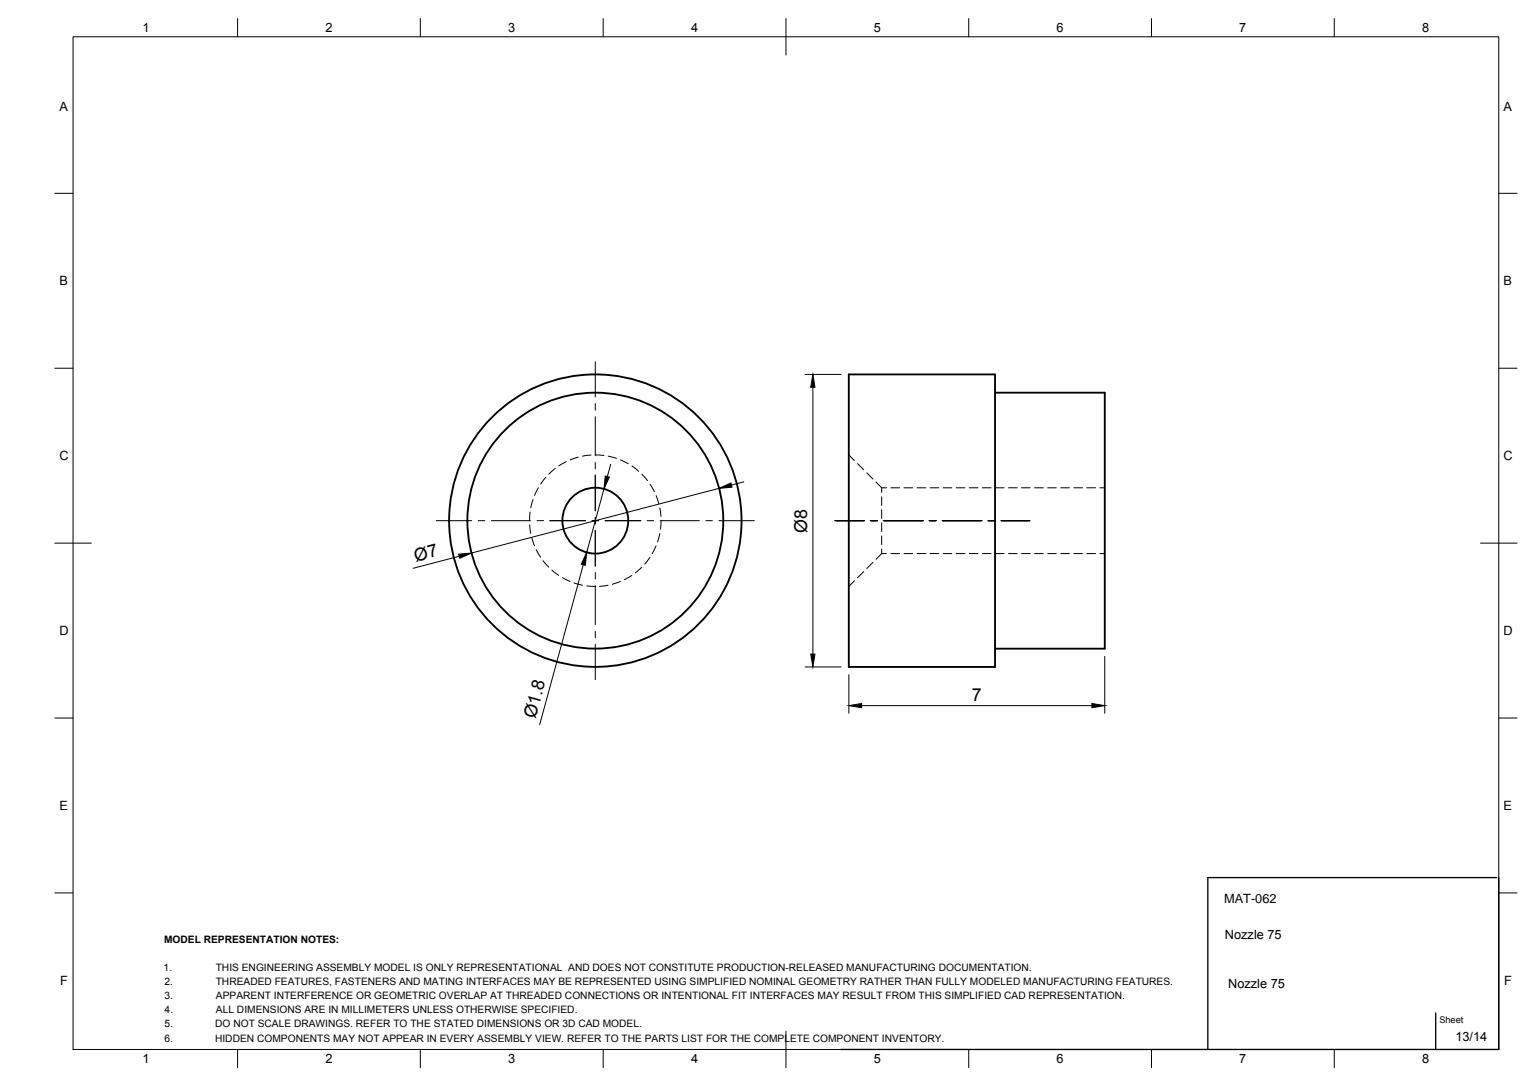
ISO-10303-21;
HEADER;
/* Generated by software containing ST-Developer
 * from STEP Tools, Inc. (www.steptools.com) 
 */

FILE_DESCRIPTION(
/* description */ (''),
/* implementation_level */ '2;1');

FILE_NAME(
/* name */ 'Nozzle 75.step',
/* time_stamp */ '2026-10-24T10:18:25-07:00',
/* author */ (''),
/* organization */ (''),
/* preprocessor_version */ 'ST-DEVELOPER v20.2',
/* originating_system */ 'Autodesk Translation Framework v15.15.0.0',
/* authorisation */ '');

FILE_SCHEMA (('AUTOMOTIVE_DESIGN { 1 0 10303 214 3 1 1 }'));
ENDSEC;

DATA;
#10=MECHANICAL_DESIGN_GEOMETRIC_PRESENTATION_REPRESENTATION('',(#262),#14125);
#196=CONICAL_SURFACE('',#6650,1.80000000000001,0.785398163397454);
#233=SHAPE_REPRESENTATION_RELATIONSHIP('SRR','None',#14207,#243);
#243=ADVANCED_BREP_SHAPE_REPRESENTATION('',(#275),#14121);
#262=STYLED_ITEM('',(#14263),#275);
#275=MANIFOLD_SOLID_BREP('Nozzle 75',#6143);
#560=CYLINDRICAL_SURFACE('',#6640,4.);
#561=CYLINDRICAL_SURFACE('',#6647,0.899999999999989);
#562=CYLINDRICAL_SURFACE('',#6653,3.49999999999993);
#681=FACE_BOUND('',#1362,.T.);
#682=FACE_BOUND('',#1364,.T.);
#683=FACE_BOUND('',#1368,.T.);
#953=FACE_OUTER_BOUND('',#1360,.T.);
#954=FACE_OUTER_BOUND('',#1361,.T.);
#955=FACE_OUTER_BOUND('',#1363,.T.);
#956=FACE_OUTER_BOUND('',#1365,.T.);
#957=FACE_OUTER_BOUND('',#1366,.T.);
#958=FACE_OUTER_BOUND('',#1367,.T.);
#959=FACE_OUTER_BOUND('',#1369,.T.);
#1360=EDGE_LOOP('',(#5025,#5026,#5027,#5028));
#1361=EDGE_LOOP('',(#5029));
#1362=EDGE_LOOP('',(#5030));
#1363=EDGE_LOOP('',(#5031));
#1364=EDGE_LOOP('',(#5032));
#1365=EDGE_LOOP('',(#5033,#5034,#5035,#5036));
#1366=EDGE_LOOP('',(#5037,#5038,#5039,#5040));
#1367=EDGE_LOOP('',(#5041));
#1368=EDGE_LOOP('',(#5042));
#1369=EDGE_LOOP('',(#5043,#5044,#5045,#5046));
#1713=CIRCLE('',#6641,4.);
#1714=CIRCLE('',#6642,4.);
#1715=CIRCLE('',#6644,3.49999999999993);
#1716=CIRCLE('',#6646,1.80000000000001);
#1717=CIRCLE('',#6648,0.900000000000014);
#1718=CIRCLE('',#6649,0.899999999999985);
#1719=CIRCLE('',#6652,3.49999999999993);
#2046=LINE('',#12270,#2434);
#2047=LINE('',#12282,#2435);
#2048=LINE('',#12285,#2436);
#2049=LINE('',#12290,#2437);
#2434=VECTOR('',#7918,4.);
#2435=VECTOR('',#7933,0.899999999999989);
#2436=VECTOR('',#7938,1.80000000000001);
#2437=VECTOR('',#7945,3.49999999999992);
#2930=VERTEX_POINT('',#12267);
#2931=VERTEX_POINT('',#12269);
#2932=VERTEX_POINT('',#12273);
#2933=VERTEX_POINT('',#12276);
#2934=VERTEX_POINT('',#12279);
#2935=VERTEX_POINT('',#12281);
#2936=VERTEX_POINT('',#12287);
#3660=EDGE_CURVE('',#2930,#2930,#1713,.T.);
#3661=EDGE_CURVE('',#2930,#2931,#2046,.T.);
#3662=EDGE_CURVE('',#2931,#2931,#1714,.T.);
#3663=EDGE_CURVE('',#2932,#2932,#1715,.T.);
#3664=EDGE_CURVE('',#2933,#2933,#1716,.T.);
#3665=EDGE_CURVE('',#2934,#2934,#1717,.T.);
#3666=EDGE_CURVE('',#2934,#2935,#2047,.T.);
#3667=EDGE_CURVE('',#2935,#2935,#1718,.T.);
#3668=EDGE_CURVE('',#2935,#2933,#2048,.T.);
#3669=EDGE_CURVE('',#2936,#2936,#1719,.T.);
#3670=EDGE_CURVE('',#2932,#2936,#2049,.T.);
#5025=ORIENTED_EDGE('',*,*,#3660,.T.);
#5026=ORIENTED_EDGE('',*,*,#3661,.T.);
#5027=ORIENTED_EDGE('',*,*,#3662,.F.);
#5028=ORIENTED_EDGE('',*,*,#3661,.F.);
#5029=ORIENTED_EDGE('',*,*,#3662,.T.);
#5030=ORIENTED_EDGE('',*,*,#3663,.F.);
#5031=ORIENTED_EDGE('',*,*,#3660,.F.);
#5032=ORIENTED_EDGE('',*,*,#3664,.F.);
#5033=ORIENTED_EDGE('',*,*,#3665,.T.);
#5034=ORIENTED_EDGE('',*,*,#3666,.T.);
#5035=ORIENTED_EDGE('',*,*,#3667,.T.);
#5036=ORIENTED_EDGE('',*,*,#3666,.F.);
#5037=ORIENTED_EDGE('',*,*,#3667,.F.);
#5038=ORIENTED_EDGE('',*,*,#3668,.T.);
#5039=ORIENTED_EDGE('',*,*,#3664,.T.);
#5040=ORIENTED_EDGE('',*,*,#3668,.F.);
#5041=ORIENTED_EDGE('',*,*,#3669,.T.);
#5042=ORIENTED_EDGE('',*,*,#3665,.F.);
#5043=ORIENTED_EDGE('',*,*,#3663,.T.);
#5044=ORIENTED_EDGE('',*,*,#3670,.T.);
#5045=ORIENTED_EDGE('',*,*,#3669,.F.);
#5046=ORIENTED_EDGE('',*,*,#3670,.F.);
#5722=PLANE('',#6643);
#5723=PLANE('',#6645);
#5724=PLANE('',#6651);
#6002=ADVANCED_FACE('',(#953),#560,.T.);
#6003=ADVANCED_FACE('',(#954,#681),#5722,.T.);
#6004=ADVANCED_FACE('',(#955,#682),#5723,.F.);
#6005=ADVANCED_FACE('',(#956),#561,.F.);
#6006=ADVANCED_FACE('',(#957),#196,.F.);
#6007=ADVANCED_FACE('',(#958,#683),#5724,.T.);
#6008=ADVANCED_FACE('',(#959),#562,.T.);
#6143=CLOSED_SHELL('',(#6002,#6003,#6004,#6005,#6006,#6007,#6008));
#6639=AXIS2_PLACEMENT_3D('',#12265,#7912,#7913);
#6640=AXIS2_PLACEMENT_3D('',#12266,#7914,#7915);
#6641=AXIS2_PLACEMENT_3D('',#12268,#7916,#7917);
#6642=AXIS2_PLACEMENT_3D('',#12271,#7919,#7920);
#6643=AXIS2_PLACEMENT_3D('',#12272,#7921,#7922);
#6644=AXIS2_PLACEMENT_3D('',#12274,#7923,#7924);
#6645=AXIS2_PLACEMENT_3D('',#12275,#7925,#7926);
#6646=AXIS2_PLACEMENT_3D('',#12277,#7927,#7928);
#6647=AXIS2_PLACEMENT_3D('',#12278,#7929,#7930);
#6648=AXIS2_PLACEMENT_3D('',#12280,#7931,#7932);
#6649=AXIS2_PLACEMENT_3D('',#12283,#7934,#7935);
#6650=AXIS2_PLACEMENT_3D('',#12284,#7936,#7937);
#6651=AXIS2_PLACEMENT_3D('',#12286,#7939,#7940);
#6652=AXIS2_PLACEMENT_3D('',#12288,#7941,#7942);
#6653=AXIS2_PLACEMENT_3D('',#12289,#7943,#7944);
#7912=DIRECTION('axis',(0.,0.,1.));
#7913=DIRECTION('refdir',(1.,0.,0.));
#7914=DIRECTION('center_axis',(-0.224143868042018,0.965925826289067,-0.129409522551263));
#7915=DIRECTION('ref_axis',(-0.974116947696296,-0.22604462437946,0.));
#7916=DIRECTION('center_axis',(0.224143868042018,-0.965925826289067,0.129409522551263));
#7917=DIRECTION('ref_axis',(0.974116947696296,0.22604462437946,0.));
#7918=DIRECTION('',(0.224143868042018,-0.965925826289067,0.129409522551263));
#7919=DIRECTION('center_axis',(0.224143868042018,-0.965925826289067,0.129409522551263));
#7920=DIRECTION('ref_axis',(0.974116947696296,0.22604462437946,0.));
#7921=DIRECTION('center_axis',(0.224143868042018,-0.965925826289067,0.129409522551263));
#7922=DIRECTION('ref_axis',(0.,-0.132788176096111,-0.991144439670156));
#7923=DIRECTION('center_axis',(0.224143868042018,-0.965925826289067,0.129409522551263));
#7924=DIRECTION('ref_axis',(0.974116947696296,0.22604462437946,0.));
#7925=DIRECTION('center_axis',(0.224143868042018,-0.965925826289067,0.129409522551263));
#7926=DIRECTION('ref_axis',(0.,-0.132788176096111,-0.991144439670156));
#7927=DIRECTION('center_axis',(-0.224143868042018,0.965925826289067,-0.129409522551263));
#7928=DIRECTION('ref_axis',(-0.974116947696296,-0.22604462437946,0.));
#7929=DIRECTION('center_axis',(-0.224143868042018,0.965925826289067,-0.129409522551263));
#7930=DIRECTION('ref_axis',(-0.974116947696296,-0.22604462437946,0.));
#7931=DIRECTION('center_axis',(0.224143868042018,-0.965925826289067,0.129409522551263));
#7932=DIRECTION('ref_axis',(0.974116947696296,0.22604462437946,0.));
#7933=DIRECTION('',(-0.224143868042018,0.965925826289067,-0.129409522551263));
#7934=DIRECTION('center_axis',(-0.224143868042018,0.965925826289067,-0.129409522551263));
#7935=DIRECTION('ref_axis',(-0.974116947696296,-0.22604462437946,0.));
#7936=DIRECTION('center_axis',(-0.224143868042018,0.965925826289067,-0.129409522551263));
#7937=DIRECTION('ref_axis',(-0.974116947696296,-0.22604462437946,0.));
#7938=DIRECTION('',(0.530311050330904,0.842850388641698,-0.091506350946111));
#7939=DIRECTION('center_axis',(0.224143868042018,-0.965925826289067,0.129409522551263));
#7940=DIRECTION('ref_axis',(0.,-0.132788176096111,-0.991144439670156));
#7941=DIRECTION('center_axis',(0.224143868042018,-0.965925826289067,0.129409522551263));
#7942=DIRECTION('ref_axis',(0.974116947696296,0.22604462437946,0.));
#7943=DIRECTION('center_axis',(-0.224143868042018,0.965925826289067,-0.129409522551263));
#7944=DIRECTION('ref_axis',(-0.974116947696296,-0.22604462437946,0.));
#7945=DIRECTION('',(0.224143868042018,-0.965925826289067,0.129409522551263));
#12265=CARTESIAN_POINT('',(0.,0.,0.));
#12266=CARTESIAN_POINT('Origin',(-88.8998569762207,131.101020514434,-63.3263563561378));
#12267=CARTESIAN_POINT('',(-85.8999646576036,135.868902317108,-63.8439944463428));
#12268=CARTESIAN_POINT('Origin',(-89.7964324483888,134.96472381959,-63.8439944463428));
#12269=CARTESIAN_POINT('',(-85.0033891854356,132.005199011951,-63.3263563561378));
#12270=CARTESIAN_POINT('',(-85.0033891854356,132.005199011951,-63.3263563561378));
#12271=CARTESIAN_POINT('Origin',(-88.8998569762207,131.101020514434,-63.3263563561378));
#12272=CARTESIAN_POINT('Origin',(-88.8998569762207,131.101020514434,-63.3263563561378));
#12273=CARTESIAN_POINT('',(-85.4904476592837,131.892176699762,-63.3263563561378));
#12274=CARTESIAN_POINT('Origin',(-88.8998569762207,131.101020514434,-63.3263563561378));
#12275=CARTESIAN_POINT('Origin',(-89.7964324483888,134.96472381959,-63.8439944463428));
#12276=CARTESIAN_POINT('',(-88.0430219425354,135.371604143473,-63.8439944463428));
#12277=CARTESIAN_POINT('Origin',(-89.7964324483888,134.96472381959,-63.8439944463428));
#12278=CARTESIAN_POINT('Origin',(-89.7964324483888,134.96472381959,-63.8439944463428));
#12279=CARTESIAN_POINT('',(-87.350720119168,128.406683197508,-62.938127788484));
#12280=CARTESIAN_POINT('Origin',(-88.2274253720946,128.203243035566,-62.938127788484));
#12281=CARTESIAN_POINT('',(-88.7179977142243,134.298830737871,-63.7275258760467));
#12282=CARTESIAN_POINT('',(-88.9197271954621,135.168163981531,-63.8439944463428));
#12283=CARTESIAN_POINT('Origin',(-89.5947029671509,134.09539057593,-63.7275258760467));
#12284=CARTESIAN_POINT('Origin',(-89.7964324483888,134.96472381959,-63.8439944463428));
#12285=CARTESIAN_POINT('',(-88.0430219425354,135.371604143473,-63.8439944463428));
#12286=CARTESIAN_POINT('Origin',(-88.2274253720946,128.203243035566,-62.938127788484));
#12287=CARTESIAN_POINT('',(-84.8180160551577,128.994399220895,-62.938127788484));
#12288=CARTESIAN_POINT('Origin',(-88.2274253720946,128.203243035566,-62.938127788484));
#12289=CARTESIAN_POINT('Origin',(-88.2274253720946,128.203243035566,-62.938127788484));
#12290=CARTESIAN_POINT('',(-84.8180160551577,128.994399220895,-62.938127788484));
#14108=UNCERTAINTY_MEASURE_WITH_UNIT(LENGTH_MEASURE(0.01),#14126,
'DISTANCE_ACCURACY_VALUE',
'Maximum model space distance between geometric entities at asserted c
onnectivities');
#14112=UNCERTAINTY_MEASURE_WITH_UNIT(LENGTH_MEASURE(0.01),#14126,
'DISTANCE_ACCURACY_VALUE',
'Maximum model space distance between geometric entities at asserted c
onnectivities');
#14121=(
GEOMETRIC_REPRESENTATION_CONTEXT(3)
GLOBAL_UNCERTAINTY_ASSIGNED_CONTEXT((#14108))
GLOBAL_UNIT_ASSIGNED_CONTEXT((#14126,#14128,#14129))
REPRESENTATION_CONTEXT('','3D')
);
#14125=(
GEOMETRIC_REPRESENTATION_CONTEXT(3)
GLOBAL_UNCERTAINTY_ASSIGNED_CONTEXT((#14112))
GLOBAL_UNIT_ASSIGNED_CONTEXT((#14126,#14128,#14129))
REPRESENTATION_CONTEXT('','3D')
);
#14126=(
LENGTH_UNIT()
NAMED_UNIT(*)
SI_UNIT(.MILLI.,.METRE.)
);
#14128=(
NAMED_UNIT(*)
PLANE_ANGLE_UNIT()
SI_UNIT($,.RADIAN.)
);
#14129=(
NAMED_UNIT(*)
SI_UNIT($,.STERADIAN.)
SOLID_ANGLE_UNIT()
);
#14138=SHAPE_DEFINITION_REPRESENTATION(#14150,#14207);
#14150=PRODUCT_DEFINITION_SHAPE('',$,#14220);
#14207=SHAPE_REPRESENTATION('',(#6639),#14121);
#14211=PRODUCT_DEFINITION_CONTEXT('part definition',#14249,'design');
#14220=PRODUCT_DEFINITION('Nozzle 75','Nozzle 75',#14232,#14211);
#14232=PRODUCT_DEFINITION_FORMATION('',$,#14259);
#14249=APPLICATION_CONTEXT(
'Core Data for Automotive Mechanical Design Process');
#14250=PRODUCT_CONTEXT('part definition',#14249,'mechanical');
#14259=PRODUCT('Nozzle 75','Nozzle 75',$,(#14250));
#14263=PRESENTATION_STYLE_ASSIGNMENT((#14265));
#14265=SURFACE_STYLE_USAGE(.BOTH.,#14267);
#14267=SURFACE_SIDE_STYLE('',(#14269));
#14269=SURFACE_STYLE_FILL_AREA(#14271);
#14271=FILL_AREA_STYLE('Steel - Satin',(#14273));
#14273=FILL_AREA_STYLE_COLOUR('Steel - Satin',#14275);
#14275=COLOUR_RGB('Steel - Satin',0.627450980392157,0.627450980392157,0.627450980392157);
ENDSEC;
END-ISO-10303-21;
